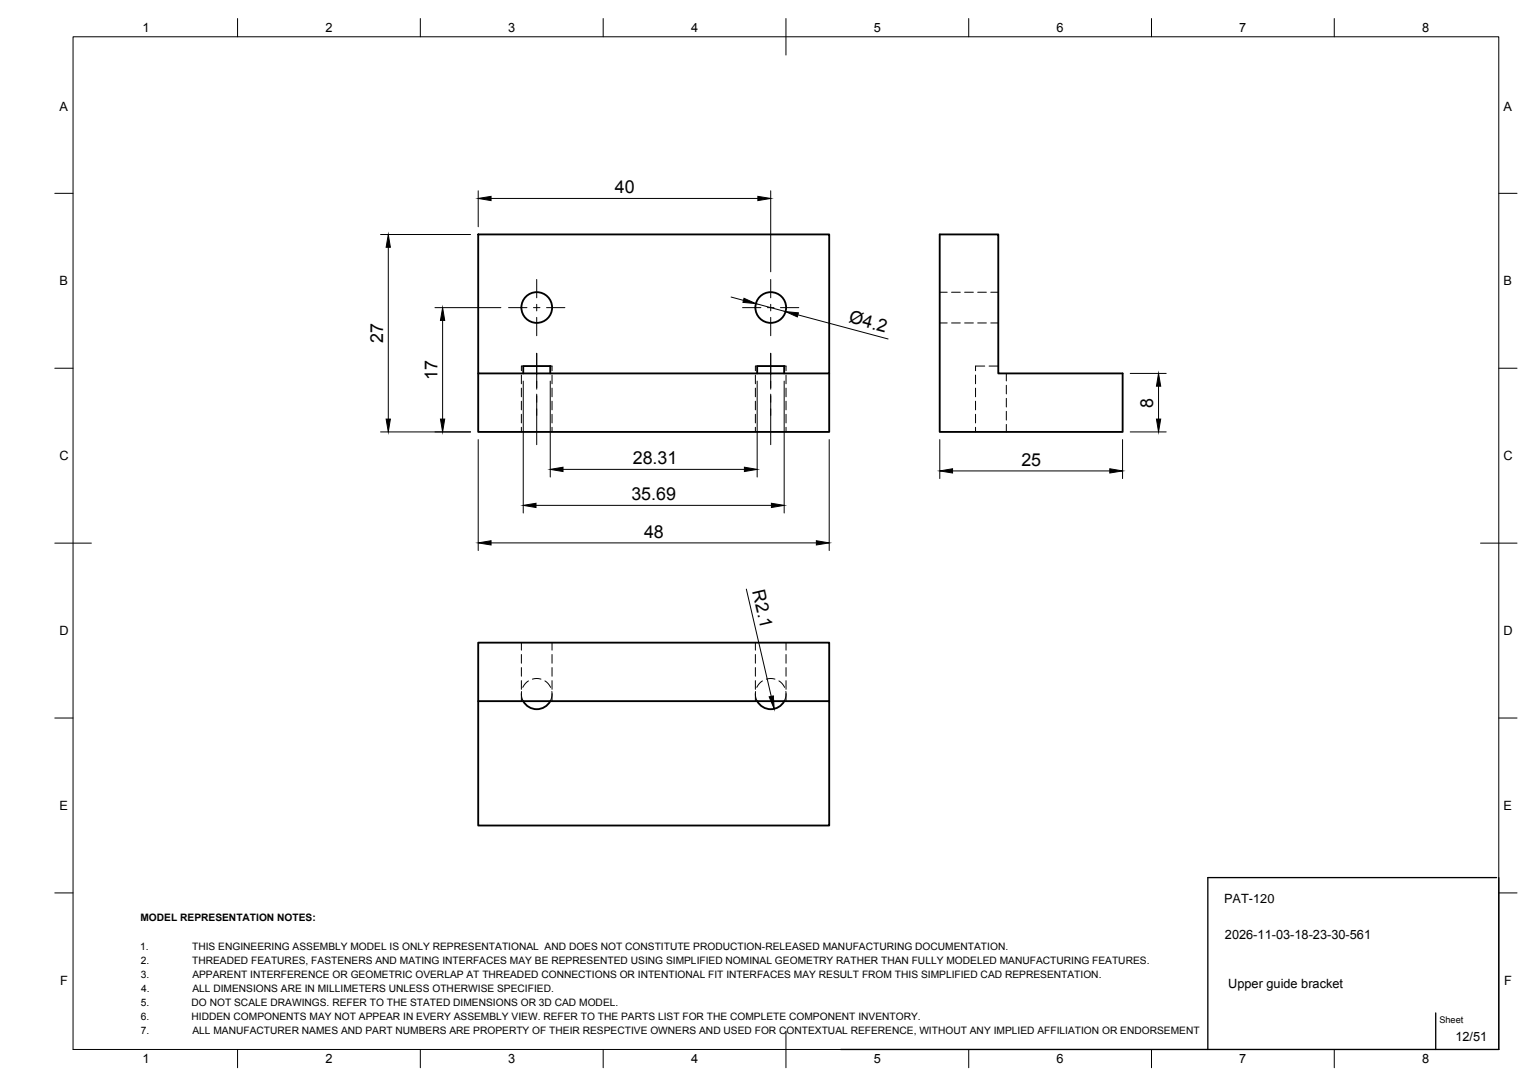
ISO-10303-21;
HEADER;
/* Generated by software containing ST-Developer
 * from STEP Tools, Inc. (www.steptools.com) 
 */

FILE_DESCRIPTION(
/* description */ ('Vibration shaker table dummy'),
/* implementation_level */ '2;1');

FILE_NAME(
/* name */ 'Upper guide bracket.step',
/* time_stamp */ '2026-10-27T10:55:14-07:00',
/* author */ (''),
/* organization */ (''),
/* preprocessor_version */ 'ST-DEVELOPER v20.2',
/* originating_system */ 'Autodesk Translation Framework v15.17.0.0',
/* authorisation */ '');

FILE_SCHEMA (('AUTOMOTIVE_DESIGN { 1 0 10303 214 3 1 1 }'));
ENDSEC;

DATA;
#10=MECHANICAL_DESIGN_GEOMETRIC_PRESENTATION_REPRESENTATION('',(#693),#22394);
#601=SHAPE_REPRESENTATION_RELATIONSHIP('SRR','None',#22647,#647);
#647=ADVANCED_BREP_SHAPE_REPRESENTATION('',(#739),#22353);
#693=STYLED_ITEM('',(#22940),#739);
#739=MANIFOLD_SOLID_BREP('Body1',#9211);
#869=FACE_BOUND('',#2045,.T.);
#870=FACE_BOUND('',#2046,.T.);
#871=FACE_BOUND('',#2050,.T.);
#872=FACE_BOUND('',#2051,.T.);
#873=FACE_BOUND('',#2054,.T.);
#874=FACE_BOUND('',#2055,.T.);
#1112=PLANE('',#9989);
#1113=PLANE('',#9995);
#1114=PLANE('',#9996);
#1115=PLANE('',#9997);
#1116=PLANE('',#9998);
#1117=PLANE('',#9999);
#1118=PLANE('',#10000);
#1119=PLANE('',#10001);
#1120=PLANE('',#10002);
#1121=PLANE('',#10003);
#1445=FACE_OUTER_BOUND('',#2037,.T.);
#1446=FACE_OUTER_BOUND('',#2038,.T.);
#1447=FACE_OUTER_BOUND('',#2039,.T.);
#1448=FACE_OUTER_BOUND('',#2040,.T.);
#1449=FACE_OUTER_BOUND('',#2041,.T.);
#1450=FACE_OUTER_BOUND('',#2042,.T.);
#1451=FACE_OUTER_BOUND('',#2043,.T.);
#1452=FACE_OUTER_BOUND('',#2044,.T.);
#1453=FACE_OUTER_BOUND('',#2047,.T.);
#1454=FACE_OUTER_BOUND('',#2048,.T.);
#1455=FACE_OUTER_BOUND('',#2049,.T.);
#1456=FACE_OUTER_BOUND('',#2052,.T.);
#1457=FACE_OUTER_BOUND('',#2053,.T.);
#1458=FACE_OUTER_BOUND('',#2056,.T.);
#2037=EDGE_LOOP('',(#6726,#6727,#6728,#6729));
#2038=EDGE_LOOP('',(#6730,#6731,#6732,#6733));
#2039=EDGE_LOOP('',(#6734,#6735,#6736,#6737,#6738,#6739,#6740,#6741));
#2040=EDGE_LOOP('',(#6742,#6743,#6744));
#2041=EDGE_LOOP('',(#6745,#6746,#6747,#6748,#6749,#6750,#6751,#6752));
#2042=EDGE_LOOP('',(#6753,#6754,#6755));
#2043=EDGE_LOOP('',(#6756,#6757,#6758,#6759,#6760,#6761,#6762,#6763));
#2044=EDGE_LOOP('',(#6764,#6765,#6766,#6767,#6768,#6769,#6770,#6771,#6772,
#6773,#6774,#6775));
#2045=EDGE_LOOP('',(#6776));
#2046=EDGE_LOOP('',(#6777));
#2047=EDGE_LOOP('',(#6778,#6779,#6780,#6781));
#2048=EDGE_LOOP('',(#6782,#6783,#6784,#6785,#6786,#6787));
#2049=EDGE_LOOP('',(#6788,#6789,#6790,#6791));
#2050=EDGE_LOOP('',(#6792));
#2051=EDGE_LOOP('',(#6793));
#2052=EDGE_LOOP('',(#6794,#6795,#6796,#6797,#6798,#6799));
#2053=EDGE_LOOP('',(#6800,#6801,#6802,#6803));
#2054=EDGE_LOOP('',(#6804));
#2055=EDGE_LOOP('',(#6805));
#2056=EDGE_LOOP('',(#6806,#6807,#6808,#6809));
#2758=LINE('',#14467,#3377);
#2759=LINE('',#14473,#3378);
#2760=LINE('',#14479,#3379);
#2761=LINE('',#14483,#3380);
#2762=LINE('',#14487,#3381);
#2763=LINE('',#14490,#3382);
#2764=LINE('',#14495,#3383);
#2765=LINE('',#14499,#3384);
#2766=LINE('',#14503,#3385);
#2767=LINE('',#14506,#3386);
#2768=LINE('',#14508,#3387);
#2769=LINE('',#14510,#3388);
#2770=LINE('',#14512,#3389);
#2771=LINE('',#14514,#3390);
#2772=LINE('',#14516,#3391);
#2773=LINE('',#14517,#3392);
#2774=LINE('',#14520,#3393);
#2775=LINE('',#14522,#3394);
#2776=LINE('',#14523,#3395);
#2777=LINE('',#14527,#3396);
#2778=LINE('',#14528,#3397);
#2779=LINE('',#14529,#3398);
#2780=LINE('',#14533,#3399);
#2781=LINE('',#14534,#3400);
#2782=LINE('',#14535,#3401);
#2783=LINE('',#14539,#3402);
#2784=LINE('',#14540,#3403);
#2785=LINE('',#14541,#3404);
#2786=LINE('',#14543,#3405);
#2787=LINE('',#14544,#3406);
#3377=VECTOR('',#11526,0.21);
#3378=VECTOR('',#11533,0.21);
#3379=VECTOR('',#11540,0.21);
#3380=VECTOR('',#11543,1.);
#3381=VECTOR('',#11546,1.);
#3382=VECTOR('',#11551,1.);
#3383=VECTOR('',#11556,0.21);
#3384=VECTOR('',#11559,1.);
#3385=VECTOR('',#11562,1.);
#3386=VECTOR('',#11567,1.);
#3387=VECTOR('',#11570,1.);
#3388=VECTOR('',#11571,1.);
#3389=VECTOR('',#11572,1.);
#3390=VECTOR('',#11573,1.);
#3391=VECTOR('',#11574,1.);
#3392=VECTOR('',#11575,1.);
#3393=VECTOR('',#11578,1.);
#3394=VECTOR('',#11579,1.);
#3395=VECTOR('',#11580,1.);
#3396=VECTOR('',#11583,1.);
#3397=VECTOR('',#11584,1.);
#3398=VECTOR('',#11585,1.);
#3399=VECTOR('',#11588,1.);
#3400=VECTOR('',#11589,1.);
#3401=VECTOR('',#11590,1.);
#3402=VECTOR('',#11593,1.);
#3403=VECTOR('',#11594,1.);
#3404=VECTOR('',#11595,1.);
#3405=VECTOR('',#11598,1.);
#3406=VECTOR('',#11599,1.);
#3964=CIRCLE('',#9979,0.21);
#3965=CIRCLE('',#9980,0.21);
#3966=CIRCLE('',#9982,0.21);
#3967=CIRCLE('',#9983,0.21);
#3968=CIRCLE('',#9985,0.21);
#3969=CIRCLE('',#9986,0.21);
#3970=CIRCLE('',#9987,0.21);
#3971=CIRCLE('',#9988,0.21);
#3972=CIRCLE('',#9991,0.21);
#3973=CIRCLE('',#9992,0.21);
#3974=CIRCLE('',#9993,0.21);
#3975=CIRCLE('',#9994,0.21);
#4527=VERTEX_POINT('',#14464);
#4528=VERTEX_POINT('',#14466);
#4529=VERTEX_POINT('',#14470);
#4530=VERTEX_POINT('',#14472);
#4531=VERTEX_POINT('',#14476);
#4532=VERTEX_POINT('',#14478);
#4533=VERTEX_POINT('',#14480);
#4534=VERTEX_POINT('',#14482);
#4535=VERTEX_POINT('',#14484);
#4536=VERTEX_POINT('',#14486);
#4537=VERTEX_POINT('',#14492);
#4538=VERTEX_POINT('',#14494);
#4539=VERTEX_POINT('',#14496);
#4540=VERTEX_POINT('',#14498);
#4541=VERTEX_POINT('',#14500);
#4542=VERTEX_POINT('',#14502);
#4543=VERTEX_POINT('',#14509);
#4544=VERTEX_POINT('',#14511);
#4545=VERTEX_POINT('',#14513);
#4546=VERTEX_POINT('',#14515);
#4547=VERTEX_POINT('',#14519);
#4548=VERTEX_POINT('',#14521);
#4549=VERTEX_POINT('',#14525);
#4550=VERTEX_POINT('',#14526);
#4551=VERTEX_POINT('',#14531);
#4552=VERTEX_POINT('',#14532);
#4553=VERTEX_POINT('',#14537);
#4554=VERTEX_POINT('',#14538);
#5356=EDGE_CURVE('',#4527,#4527,#3964,.T.);
#5357=EDGE_CURVE('',#4527,#4528,#2758,.T.);
#5358=EDGE_CURVE('',#4528,#4528,#3965,.T.);
#5359=EDGE_CURVE('',#4529,#4529,#3966,.T.);
#5360=EDGE_CURVE('',#4529,#4530,#2759,.T.);
#5361=EDGE_CURVE('',#4530,#4530,#3967,.T.);
#5362=EDGE_CURVE('',#4531,#4531,#3968,.T.);
#5363=EDGE_CURVE('',#4531,#4532,#2760,.T.);
#5364=EDGE_CURVE('',#4532,#4533,#3969,.T.);
#5365=EDGE_CURVE('',#4534,#4533,#2761,.T.);
#5366=EDGE_CURVE('',#4535,#4534,#3970,.T.);
#5367=EDGE_CURVE('',#4536,#4535,#2762,.T.);
#5368=EDGE_CURVE('',#4536,#4532,#3971,.T.);
#5369=EDGE_CURVE('',#4533,#4536,#2763,.T.);
#5370=EDGE_CURVE('',#4537,#4537,#3972,.T.);
#5371=EDGE_CURVE('',#4537,#4538,#2764,.T.);
#5372=EDGE_CURVE('',#4538,#4539,#3973,.T.);
#5373=EDGE_CURVE('',#4540,#4539,#2765,.T.);
#5374=EDGE_CURVE('',#4541,#4540,#3974,.T.);
#5375=EDGE_CURVE('',#4542,#4541,#2766,.T.);
#5376=EDGE_CURVE('',#4542,#4538,#3975,.T.);
#5377=EDGE_CURVE('',#4539,#4542,#2767,.T.);
#5378=EDGE_CURVE('',#4534,#4541,#2768,.T.);
#5379=EDGE_CURVE('',#4540,#4543,#2769,.T.);
#5380=EDGE_CURVE('',#4544,#4543,#2770,.T.);
#5381=EDGE_CURVE('',#4544,#4545,#2771,.T.);
#5382=EDGE_CURVE('',#4545,#4546,#2772,.T.);
#5383=EDGE_CURVE('',#4546,#4535,#2773,.T.);
#5384=EDGE_CURVE('',#4546,#4547,#2774,.T.);
#5385=EDGE_CURVE('',#4548,#4547,#2775,.T.);
#5386=EDGE_CURVE('',#4543,#4548,#2776,.T.);
#5387=EDGE_CURVE('',#4549,#4550,#2777,.T.);
#5388=EDGE_CURVE('',#4550,#4548,#2778,.T.);
#5389=EDGE_CURVE('',#4547,#4549,#2779,.T.);
#5390=EDGE_CURVE('',#4551,#4552,#2780,.T.);
#5391=EDGE_CURVE('',#4551,#4544,#2781,.T.);
#5392=EDGE_CURVE('',#4552,#4550,#2782,.T.);
#5393=EDGE_CURVE('',#4553,#4554,#2783,.T.);
#5394=EDGE_CURVE('',#4553,#4551,#2784,.T.);
#5395=EDGE_CURVE('',#4554,#4552,#2785,.T.);
#5396=EDGE_CURVE('',#4545,#4553,#2786,.T.);
#5397=EDGE_CURVE('',#4554,#4549,#2787,.T.);
#6726=ORIENTED_EDGE('',*,*,#5356,.F.);
#6727=ORIENTED_EDGE('',*,*,#5357,.T.);
#6728=ORIENTED_EDGE('',*,*,#5358,.F.);
#6729=ORIENTED_EDGE('',*,*,#5357,.F.);
#6730=ORIENTED_EDGE('',*,*,#5359,.F.);
#6731=ORIENTED_EDGE('',*,*,#5360,.T.);
#6732=ORIENTED_EDGE('',*,*,#5361,.F.);
#6733=ORIENTED_EDGE('',*,*,#5360,.F.);
#6734=ORIENTED_EDGE('',*,*,#5362,.F.);
#6735=ORIENTED_EDGE('',*,*,#5363,.T.);
#6736=ORIENTED_EDGE('',*,*,#5364,.T.);
#6737=ORIENTED_EDGE('',*,*,#5365,.F.);
#6738=ORIENTED_EDGE('',*,*,#5366,.F.);
#6739=ORIENTED_EDGE('',*,*,#5367,.F.);
#6740=ORIENTED_EDGE('',*,*,#5368,.T.);
#6741=ORIENTED_EDGE('',*,*,#5363,.F.);
#6742=ORIENTED_EDGE('',*,*,#5369,.F.);
#6743=ORIENTED_EDGE('',*,*,#5364,.F.);
#6744=ORIENTED_EDGE('',*,*,#5368,.F.);
#6745=ORIENTED_EDGE('',*,*,#5370,.F.);
#6746=ORIENTED_EDGE('',*,*,#5371,.T.);
#6747=ORIENTED_EDGE('',*,*,#5372,.T.);
#6748=ORIENTED_EDGE('',*,*,#5373,.F.);
#6749=ORIENTED_EDGE('',*,*,#5374,.F.);
#6750=ORIENTED_EDGE('',*,*,#5375,.F.);
#6751=ORIENTED_EDGE('',*,*,#5376,.T.);
#6752=ORIENTED_EDGE('',*,*,#5371,.F.);
#6753=ORIENTED_EDGE('',*,*,#5377,.F.);
#6754=ORIENTED_EDGE('',*,*,#5372,.F.);
#6755=ORIENTED_EDGE('',*,*,#5376,.F.);
#6756=ORIENTED_EDGE('',*,*,#5366,.T.);
#6757=ORIENTED_EDGE('',*,*,#5378,.T.);
#6758=ORIENTED_EDGE('',*,*,#5374,.T.);
#6759=ORIENTED_EDGE('',*,*,#5379,.T.);
#6760=ORIENTED_EDGE('',*,*,#5380,.F.);
#6761=ORIENTED_EDGE('',*,*,#5381,.T.);
#6762=ORIENTED_EDGE('',*,*,#5382,.T.);
#6763=ORIENTED_EDGE('',*,*,#5383,.T.);
#6764=ORIENTED_EDGE('',*,*,#5367,.T.);
#6765=ORIENTED_EDGE('',*,*,#5383,.F.);
#6766=ORIENTED_EDGE('',*,*,#5384,.T.);
#6767=ORIENTED_EDGE('',*,*,#5385,.F.);
#6768=ORIENTED_EDGE('',*,*,#5386,.F.);
#6769=ORIENTED_EDGE('',*,*,#5379,.F.);
#6770=ORIENTED_EDGE('',*,*,#5373,.T.);
#6771=ORIENTED_EDGE('',*,*,#5377,.T.);
#6772=ORIENTED_EDGE('',*,*,#5375,.T.);
#6773=ORIENTED_EDGE('',*,*,#5378,.F.);
#6774=ORIENTED_EDGE('',*,*,#5365,.T.);
#6775=ORIENTED_EDGE('',*,*,#5369,.T.);
#6776=ORIENTED_EDGE('',*,*,#5356,.T.);
#6777=ORIENTED_EDGE('',*,*,#5359,.T.);
#6778=ORIENTED_EDGE('',*,*,#5387,.T.);
#6779=ORIENTED_EDGE('',*,*,#5388,.T.);
#6780=ORIENTED_EDGE('',*,*,#5385,.T.);
#6781=ORIENTED_EDGE('',*,*,#5389,.T.);
#6782=ORIENTED_EDGE('',*,*,#5390,.F.);
#6783=ORIENTED_EDGE('',*,*,#5391,.T.);
#6784=ORIENTED_EDGE('',*,*,#5380,.T.);
#6785=ORIENTED_EDGE('',*,*,#5386,.T.);
#6786=ORIENTED_EDGE('',*,*,#5388,.F.);
#6787=ORIENTED_EDGE('',*,*,#5392,.F.);
#6788=ORIENTED_EDGE('',*,*,#5393,.F.);
#6789=ORIENTED_EDGE('',*,*,#5394,.T.);
#6790=ORIENTED_EDGE('',*,*,#5390,.T.);
#6791=ORIENTED_EDGE('',*,*,#5395,.F.);
#6792=ORIENTED_EDGE('',*,*,#5362,.T.);
#6793=ORIENTED_EDGE('',*,*,#5370,.T.);
#6794=ORIENTED_EDGE('',*,*,#5382,.F.);
#6795=ORIENTED_EDGE('',*,*,#5396,.T.);
#6796=ORIENTED_EDGE('',*,*,#5393,.T.);
#6797=ORIENTED_EDGE('',*,*,#5397,.T.);
#6798=ORIENTED_EDGE('',*,*,#5389,.F.);
#6799=ORIENTED_EDGE('',*,*,#5384,.F.);
#6800=ORIENTED_EDGE('',*,*,#5397,.F.);
#6801=ORIENTED_EDGE('',*,*,#5395,.T.);
#6802=ORIENTED_EDGE('',*,*,#5392,.T.);
#6803=ORIENTED_EDGE('',*,*,#5387,.F.);
#6804=ORIENTED_EDGE('',*,*,#5358,.T.);
#6805=ORIENTED_EDGE('',*,*,#5361,.T.);
#6806=ORIENTED_EDGE('',*,*,#5396,.F.);
#6807=ORIENTED_EDGE('',*,*,#5381,.F.);
#6808=ORIENTED_EDGE('',*,*,#5391,.F.);
#6809=ORIENTED_EDGE('',*,*,#5394,.F.);
#8558=CYLINDRICAL_SURFACE('',#9978,0.21);
#8559=CYLINDRICAL_SURFACE('',#9981,0.21);
#8560=CYLINDRICAL_SURFACE('',#9984,0.21);
#8561=CYLINDRICAL_SURFACE('',#9990,0.21);
#8810=ADVANCED_FACE('',(#1445),#8558,.F.);
#8811=ADVANCED_FACE('',(#1446),#8559,.F.);
#8812=ADVANCED_FACE('',(#1447),#8560,.F.);
#8813=ADVANCED_FACE('',(#1448),#1112,.F.);
#8814=ADVANCED_FACE('',(#1449),#8561,.F.);
#8815=ADVANCED_FACE('',(#1450),#1113,.F.);
#8816=ADVANCED_FACE('',(#1451),#1114,.T.);
#8817=ADVANCED_FACE('',(#1452,#869,#870),#1115,.T.);
#8818=ADVANCED_FACE('',(#1453),#1116,.T.);
#8819=ADVANCED_FACE('',(#1454),#1117,.T.);
#8820=ADVANCED_FACE('',(#1455,#871,#872),#1118,.T.);
#8821=ADVANCED_FACE('',(#1456),#1119,.T.);
#8822=ADVANCED_FACE('',(#1457,#873,#874),#1120,.T.);
#8823=ADVANCED_FACE('',(#1458),#1121,.F.);
#9211=CLOSED_SHELL('',(#8810,#8811,#8812,#8813,#8814,#8815,#8816,#8817,
#8818,#8819,#8820,#8821,#8822,#8823));
#9977=AXIS2_PLACEMENT_3D('',#14462,#11520,#11521);
#9978=AXIS2_PLACEMENT_3D('',#14463,#11522,#11523);
#9979=AXIS2_PLACEMENT_3D('',#14465,#11524,#11525);
#9980=AXIS2_PLACEMENT_3D('',#14468,#11527,#11528);
#9981=AXIS2_PLACEMENT_3D('',#14469,#11529,#11530);
#9982=AXIS2_PLACEMENT_3D('',#14471,#11531,#11532);
#9983=AXIS2_PLACEMENT_3D('',#14474,#11534,#11535);
#9984=AXIS2_PLACEMENT_3D('',#14475,#11536,#11537);
#9985=AXIS2_PLACEMENT_3D('',#14477,#11538,#11539);
#9986=AXIS2_PLACEMENT_3D('',#14481,#11541,#11542);
#9987=AXIS2_PLACEMENT_3D('',#14485,#11544,#11545);
#9988=AXIS2_PLACEMENT_3D('',#14488,#11547,#11548);
#9989=AXIS2_PLACEMENT_3D('',#14489,#11549,#11550);
#9990=AXIS2_PLACEMENT_3D('',#14491,#11552,#11553);
#9991=AXIS2_PLACEMENT_3D('',#14493,#11554,#11555);
#9992=AXIS2_PLACEMENT_3D('',#14497,#11557,#11558);
#9993=AXIS2_PLACEMENT_3D('',#14501,#11560,#11561);
#9994=AXIS2_PLACEMENT_3D('',#14504,#11563,#11564);
#9995=AXIS2_PLACEMENT_3D('',#14505,#11565,#11566);
#9996=AXIS2_PLACEMENT_3D('',#14507,#11568,#11569);
#9997=AXIS2_PLACEMENT_3D('',#14518,#11576,#11577);
#9998=AXIS2_PLACEMENT_3D('',#14524,#11581,#11582);
#9999=AXIS2_PLACEMENT_3D('',#14530,#11586,#11587);
#10000=AXIS2_PLACEMENT_3D('',#14536,#11591,#11592);
#10001=AXIS2_PLACEMENT_3D('',#14542,#11596,#11597);
#10002=AXIS2_PLACEMENT_3D('',#14545,#11600,#11601);
#10003=AXIS2_PLACEMENT_3D('',#14546,#11602,#11603);
#11520=DIRECTION('axis',(0.,0.,1.));
#11521=DIRECTION('refdir',(1.,0.,0.));
#11522=DIRECTION('center_axis',(0.,0.,1.));
#11523=DIRECTION('ref_axis',(1.,0.,0.));
#11524=DIRECTION('center_axis',(0.,0.,1.));
#11525=DIRECTION('ref_axis',(1.,0.,0.));
#11526=DIRECTION('',(0.,0.,1.));
#11527=DIRECTION('center_axis',(0.,0.,-1.));
#11528=DIRECTION('ref_axis',(1.,0.,0.));
#11529=DIRECTION('center_axis',(0.,0.,1.));
#11530=DIRECTION('ref_axis',(1.,0.,0.));
#11531=DIRECTION('center_axis',(0.,0.,1.));
#11532=DIRECTION('ref_axis',(1.,0.,0.));
#11533=DIRECTION('',(0.,0.,1.));
#11534=DIRECTION('center_axis',(0.,0.,-1.));
#11535=DIRECTION('ref_axis',(1.,0.,0.));
#11536=DIRECTION('center_axis',(0.,1.,0.));
#11537=DIRECTION('ref_axis',(1.,0.,0.));
#11538=DIRECTION('center_axis',(0.,1.,0.));
#11539=DIRECTION('ref_axis',(1.,0.,0.));
#11540=DIRECTION('',(0.,1.,0.));
#11541=DIRECTION('center_axis',(0.,1.,0.));
#11542=DIRECTION('ref_axis',(1.,0.,0.));
#11543=DIRECTION('',(0.,1.,0.));
#11544=DIRECTION('center_axis',(0.,-1.,0.));
#11545=DIRECTION('ref_axis',(1.,0.,0.));
#11546=DIRECTION('',(0.,-1.,0.));
#11547=DIRECTION('center_axis',(0.,1.,0.));
#11548=DIRECTION('ref_axis',(1.,0.,0.));
#11549=DIRECTION('center_axis',(0.,1.,0.));
#11550=DIRECTION('ref_axis',(1.,0.,0.));
#11551=DIRECTION('',(-1.,0.,0.));
#11552=DIRECTION('center_axis',(0.,1.,0.));
#11553=DIRECTION('ref_axis',(1.,0.,0.));
#11554=DIRECTION('center_axis',(0.,1.,0.));
#11555=DIRECTION('ref_axis',(1.,0.,0.));
#11556=DIRECTION('',(0.,1.,0.));
#11557=DIRECTION('center_axis',(0.,1.,0.));
#11558=DIRECTION('ref_axis',(1.,0.,0.));
#11559=DIRECTION('',(0.,1.,0.));
#11560=DIRECTION('center_axis',(0.,-1.,0.));
#11561=DIRECTION('ref_axis',(1.,0.,0.));
#11562=DIRECTION('',(0.,-1.,0.));
#11563=DIRECTION('center_axis',(0.,1.,0.));
#11564=DIRECTION('ref_axis',(1.,0.,0.));
#11565=DIRECTION('center_axis',(0.,1.,0.));
#11566=DIRECTION('ref_axis',(1.,0.,0.));
#11567=DIRECTION('',(-1.,0.,0.));
#11568=DIRECTION('center_axis',(0.,1.,0.));
#11569=DIRECTION('ref_axis',(-1.,0.,0.));
#11570=DIRECTION('',(1.,0.,0.));
#11571=DIRECTION('',(1.,0.,0.));
#11572=DIRECTION('',(0.,0.,1.));
#11573=DIRECTION('',(-1.,0.,0.));
#11574=DIRECTION('',(0.,0.,1.));
#11575=DIRECTION('',(1.,0.,0.));
#11576=DIRECTION('center_axis',(0.,0.,-1.));
#11577=DIRECTION('ref_axis',(-1.,0.,0.));
#11578=DIRECTION('',(0.,1.,0.));
#11579=DIRECTION('',(-1.,0.,0.));
#11580=DIRECTION('',(0.,1.,0.));
#11581=DIRECTION('center_axis',(0.,1.,0.));
#11582=DIRECTION('ref_axis',(0.,0.,1.));
#11583=DIRECTION('',(1.,0.,0.));
#11584=DIRECTION('',(0.,0.,-1.));
#11585=DIRECTION('',(0.,0.,1.));
#11586=DIRECTION('center_axis',(1.,0.,0.));
#11587=DIRECTION('ref_axis',(0.,1.,0.));
#11588=DIRECTION('',(0.,0.,1.));
#11589=DIRECTION('',(0.,1.,0.));
#11590=DIRECTION('',(0.,1.,0.));
#11591=DIRECTION('center_axis',(0.,-1.,0.));
#11592=DIRECTION('ref_axis',(1.,0.,0.));
#11593=DIRECTION('',(0.,0.,1.));
#11594=DIRECTION('',(1.,0.,0.));
#11595=DIRECTION('',(1.,0.,0.));
#11596=DIRECTION('center_axis',(-1.,0.,0.));
#11597=DIRECTION('ref_axis',(0.,-1.,0.));
#11598=DIRECTION('',(0.,-1.,0.));
#11599=DIRECTION('',(0.,1.,0.));
#11600=DIRECTION('center_axis',(0.,0.,1.));
#11601=DIRECTION('ref_axis',(1.,0.,0.));
#11602=DIRECTION('center_axis',(0.,0.,1.));
#11603=DIRECTION('ref_axis',(1.,0.,0.));
#14462=CARTESIAN_POINT('',(0.,0.,0.));
#14463=CARTESIAN_POINT('Origin',(-7.6,0.,29.6));
#14464=CARTESIAN_POINT('',(-7.81,-2.57175827820944E-17,29.7));
#14465=CARTESIAN_POINT('Origin',(-7.6,0.,29.7));
#14466=CARTESIAN_POINT('',(-7.81,2.57175827820944E-17,30.5));
#14467=CARTESIAN_POINT('',(-7.81,-2.57175827820944E-17,29.6));
#14468=CARTESIAN_POINT('Origin',(-7.6,0.,30.5));
#14469=CARTESIAN_POINT('Origin',(-4.4,0.,29.6));
#14470=CARTESIAN_POINT('',(-4.61,-2.57175827820944E-17,29.7));
#14471=CARTESIAN_POINT('Origin',(-4.4,0.,29.7));
#14472=CARTESIAN_POINT('',(-4.61,2.57175827820944E-17,30.5));
#14473=CARTESIAN_POINT('',(-4.61,-2.57175827820944E-17,29.6));
#14474=CARTESIAN_POINT('Origin',(-4.4,0.,30.5));
#14475=CARTESIAN_POINT('Origin',(-7.6,-1.8,29.8));
#14476=CARTESIAN_POINT('',(-7.81,-1.7,29.8));
#14477=CARTESIAN_POINT('Origin',(-7.6,-1.7,29.8));
#14478=CARTESIAN_POINT('',(-7.81,-0.8,29.8));
#14479=CARTESIAN_POINT('',(-7.81,-1.8,29.8));
#14480=CARTESIAN_POINT('',(-7.41533814687381,-0.8,29.7));
#14481=CARTESIAN_POINT('Origin',(-7.6,-0.8,29.8));
#14482=CARTESIAN_POINT('',(-7.4153381468738,-0.9,29.7));
#14483=CARTESIAN_POINT('',(-7.41533814687381,-1.8,29.7));
#14484=CARTESIAN_POINT('',(-7.78466185312619,-0.9,29.7));
#14485=CARTESIAN_POINT('Origin',(-7.6,-0.9,29.8));
#14486=CARTESIAN_POINT('',(-7.78466185312619,-0.8,29.7));
#14487=CARTESIAN_POINT('',(-7.78466185312619,-1.8,29.7));
#14488=CARTESIAN_POINT('Origin',(-7.6,-0.8,29.8));
#14489=CARTESIAN_POINT('Origin',(-7.6,-0.8,29.8));
#14490=CARTESIAN_POINT('',(-5.6,-0.8,29.7));
#14491=CARTESIAN_POINT('Origin',(-4.4,-1.8,29.8));
#14492=CARTESIAN_POINT('',(-4.61,-1.7,29.8));
#14493=CARTESIAN_POINT('Origin',(-4.4,-1.7,29.8));
#14494=CARTESIAN_POINT('',(-4.61,-0.8,29.8));
#14495=CARTESIAN_POINT('',(-4.61,-1.8,29.8));
#14496=CARTESIAN_POINT('',(-4.21533814687381,-0.8,29.7));
#14497=CARTESIAN_POINT('Origin',(-4.4,-0.8,29.8));
#14498=CARTESIAN_POINT('',(-4.21533814687381,-0.9,29.7));
#14499=CARTESIAN_POINT('',(-4.21533814687381,-1.8,29.7));
#14500=CARTESIAN_POINT('',(-4.5846618531262,-0.9,29.7));
#14501=CARTESIAN_POINT('Origin',(-4.4,-0.9,29.8));
#14502=CARTESIAN_POINT('',(-4.58466185312619,-0.8,29.7));
#14503=CARTESIAN_POINT('',(-4.58466185312619,-1.8,29.7));
#14504=CARTESIAN_POINT('Origin',(-4.4,-0.8,29.8));
#14505=CARTESIAN_POINT('Origin',(-4.4,-0.8,29.8));
#14506=CARTESIAN_POINT('',(-4.,-0.8,29.7));
#14507=CARTESIAN_POINT('Origin',(-3.6,-0.9,28.));
#14508=CARTESIAN_POINT('',(-3.6,-0.9,29.7));
#14509=CARTESIAN_POINT('',(-3.6,-0.9,29.7));
#14510=CARTESIAN_POINT('',(-3.6,-0.9,29.7));
#14511=CARTESIAN_POINT('',(-3.6,-0.9,28.));
#14512=CARTESIAN_POINT('',(-3.6,-0.9,28.));
#14513=CARTESIAN_POINT('',(-8.4,-0.9,28.));
#14514=CARTESIAN_POINT('',(-3.6,-0.9,28.));
#14515=CARTESIAN_POINT('',(-8.4,-0.9,29.7));
#14516=CARTESIAN_POINT('',(-8.4,-0.9,28.));
#14517=CARTESIAN_POINT('',(-3.6,-0.9,29.7));
#14518=CARTESIAN_POINT('Origin',(-3.6,-1.7,29.7));
#14519=CARTESIAN_POINT('',(-8.4,1.,29.7));
#14520=CARTESIAN_POINT('',(-8.4,-1.7,29.7));
#14521=CARTESIAN_POINT('',(-3.6,1.,29.7));
#14522=CARTESIAN_POINT('',(-8.4,1.,29.7));
#14523=CARTESIAN_POINT('',(-3.6,-1.7,29.7));
#14524=CARTESIAN_POINT('Origin',(-6.,1.,30.1));
#14525=CARTESIAN_POINT('',(-8.4,1.,30.5));
#14526=CARTESIAN_POINT('',(-3.6,1.,30.5));
#14527=CARTESIAN_POINT('',(-3.6,1.,30.5));
#14528=CARTESIAN_POINT('',(-3.6,1.,29.7));
#14529=CARTESIAN_POINT('',(-8.4,1.,30.5));
#14530=CARTESIAN_POINT('Origin',(-3.6,-1.7,28.));
#14531=CARTESIAN_POINT('',(-3.6,-1.7,28.));
#14532=CARTESIAN_POINT('',(-3.6,-1.7,30.5));
#14533=CARTESIAN_POINT('',(-3.6,-1.7,28.));
#14534=CARTESIAN_POINT('',(-3.6,-1.7,28.));
#14535=CARTESIAN_POINT('',(-3.6,-1.7,30.5));
#14536=CARTESIAN_POINT('Origin',(-8.4,-1.7,28.));
#14537=CARTESIAN_POINT('',(-8.4,-1.7,28.));
#14538=CARTESIAN_POINT('',(-8.4,-1.7,30.5));
#14539=CARTESIAN_POINT('',(-8.4,-1.7,28.));
#14540=CARTESIAN_POINT('',(-8.4,-1.7,28.));
#14541=CARTESIAN_POINT('',(-8.4,-1.7,30.5));
#14542=CARTESIAN_POINT('Origin',(-8.4,-0.9,28.));
#14543=CARTESIAN_POINT('',(-8.4,-0.9,28.));
#14544=CARTESIAN_POINT('',(-8.4,-1.7,30.5));
#14545=CARTESIAN_POINT('Origin',(-6.,-1.3,30.5));
#14546=CARTESIAN_POINT('Origin',(-6.,-1.3,28.));
#22302=UNCERTAINTY_MEASURE_WITH_UNIT(LENGTH_MEASURE(0.001),#22395,
'DISTANCE_ACCURACY_VALUE',
'Maximum model space distance between geometric entities at asserted c
onnectivities');
#22343=UNCERTAINTY_MEASURE_WITH_UNIT(LENGTH_MEASURE(0.001),#22395,
'DISTANCE_ACCURACY_VALUE',
'Maximum model space distance between geometric entities at asserted c
onnectivities');
#22353=(
GEOMETRIC_REPRESENTATION_CONTEXT(3)
GLOBAL_UNCERTAINTY_ASSIGNED_CONTEXT((#22302))
GLOBAL_UNIT_ASSIGNED_CONTEXT((#22395,#22397,#22398))
REPRESENTATION_CONTEXT('','3D')
);
#22394=(
GEOMETRIC_REPRESENTATION_CONTEXT(3)
GLOBAL_UNCERTAINTY_ASSIGNED_CONTEXT((#22343))
GLOBAL_UNIT_ASSIGNED_CONTEXT((#22395,#22397,#22398))
REPRESENTATION_CONTEXT('','3D')
);
#22395=(
LENGTH_UNIT()
NAMED_UNIT(*)
SI_UNIT(.CENTI.,.METRE.)
);
#22397=(
NAMED_UNIT(*)
PLANE_ANGLE_UNIT()
SI_UNIT($,.RADIAN.)
);
#22398=(
NAMED_UNIT(*)
SI_UNIT($,.STERADIAN.)
SOLID_ANGLE_UNIT()
);
#22408=SHAPE_DEFINITION_REPRESENTATION(#22458,#22647);
#22458=PRODUCT_DEFINITION_SHAPE('',$,#22698);
#22647=SHAPE_REPRESENTATION('',(#9977),#22353);
#22688=PRODUCT_DEFINITION_CONTEXT('part definition',#22840,'design');
#22698=PRODUCT_DEFINITION('Upper guide bracket','Upper guide bracket',#22748,
#22688);
#22748=PRODUCT_DEFINITION_FORMATION('',$,#22851);
#22840=APPLICATION_CONTEXT(
'Core Data for Automotive Mechanical Design Process');
#22841=PRODUCT_CONTEXT('part definition',#22840,'mechanical');
#22851=PRODUCT('Upper guide bracket','Upper guide bracket',
'Upper guide bracket',(#22841));
#22934=COLOUR_RGB('Dark Blue',0.08,0.2,0.34);
#22935=FILL_AREA_STYLE_COLOUR('',#22934);
#22936=FILL_AREA_STYLE('',(#22935));
#22937=SURFACE_STYLE_FILL_AREA(#22936);
#22938=SURFACE_SIDE_STYLE('',(#22937));
#22939=SURFACE_STYLE_USAGE(.BOTH.,#22938);
#22940=PRESENTATION_STYLE_ASSIGNMENT((#22939));
ENDSEC;
END-ISO-10303-21;
